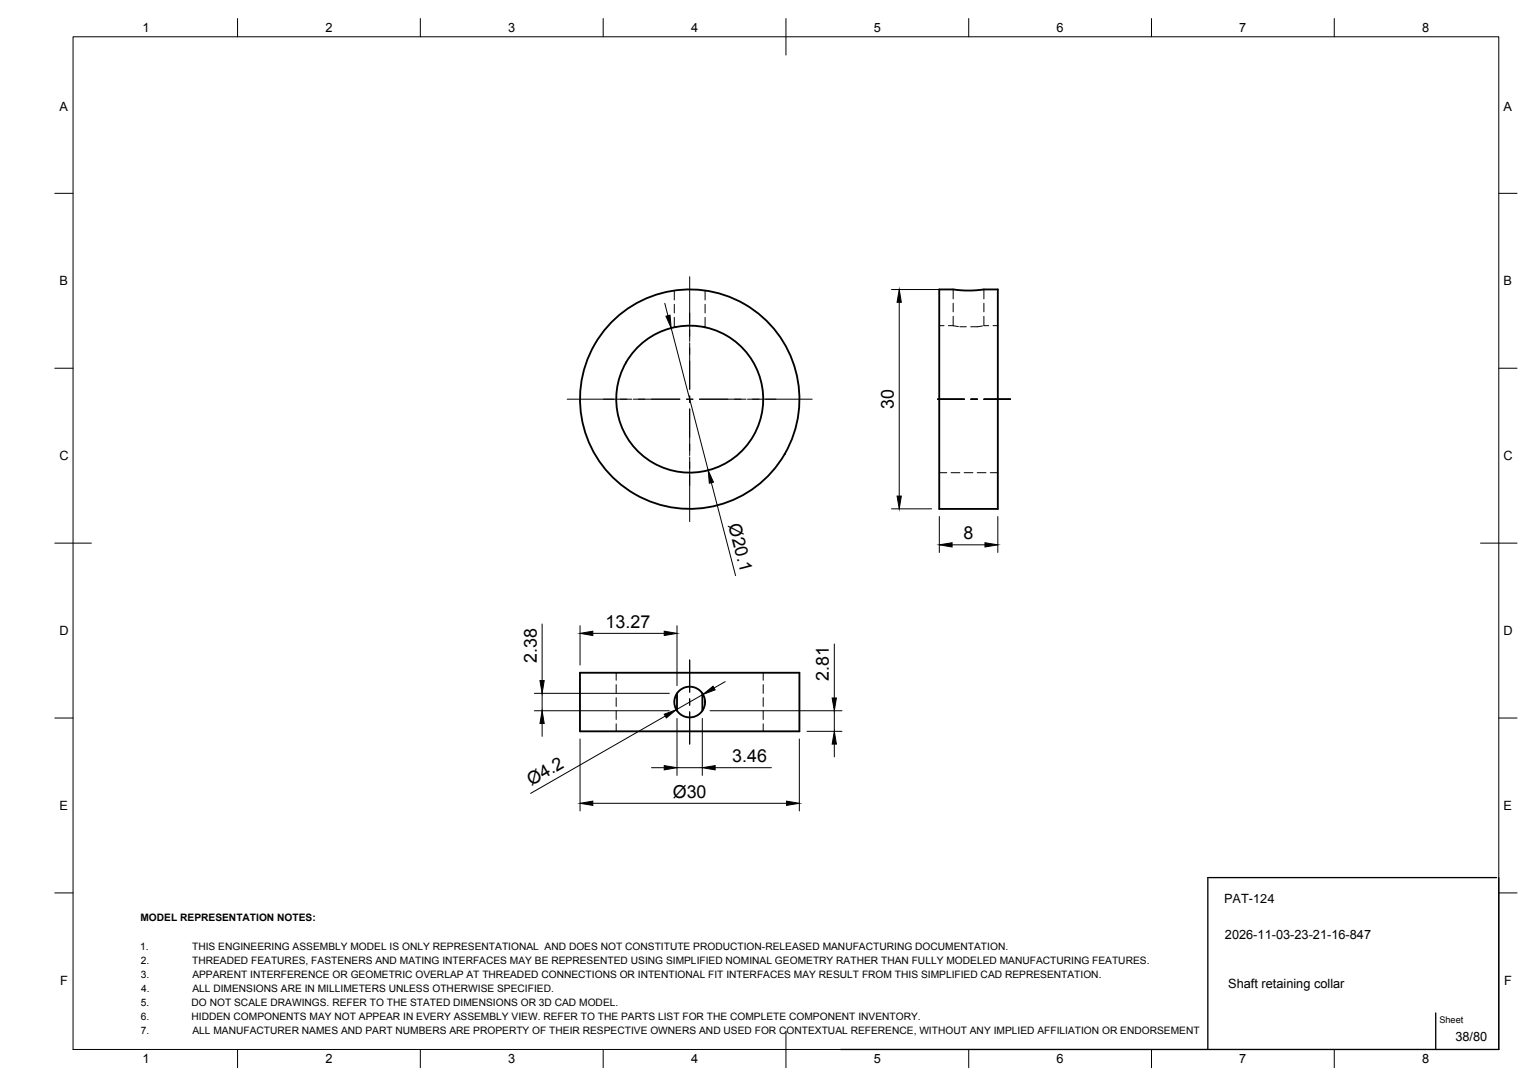
ISO-10303-21;
HEADER;
/* Generated by software containing ST-Developer
 * from STEP Tools, Inc. (www.steptools.com) 
 */

FILE_DESCRIPTION(
/* description */ ('XY cross-slide table'),
/* implementation_level */ '2;1');

FILE_NAME(
/* name */ 'Shaft retaining collar.step',
/* time_stamp */ '2026-10-28T03:22:46-07:00',
/* author */ (''),
/* organization */ (''),
/* preprocessor_version */ 'ST-DEVELOPER v20.2',
/* originating_system */ 'Autodesk Translation Framework v15.17.0.0',
/* authorisation */ '');

FILE_SCHEMA (('AUTOMOTIVE_DESIGN { 1 0 10303 214 3 1 1 }'));
ENDSEC;

DATA;
#10=MECHANICAL_DESIGN_GEOMETRIC_PRESENTATION_REPRESENTATION('',(#1719),#62984);
#1027=B_SPLINE_CURVE_WITH_KNOTS('',3,(#47301,#47302,#47303,#47304,#47305,
#47306,#47307,#47308),.UNSPECIFIED.,.F.,.F.,(4,2,2,4),(0.756005737987019,
0.793568827564653,0.872922520054208,0.952276212543762),.UNSPECIFIED.);
#1028=B_SPLINE_CURVE_WITH_KNOTS('',3,(#47311,#47312,#47313,#47314,#47315,
#47316,#47317,#47318,#47319,#47320,#47321,#47322,#47323,#47324),
 .UNSPECIFIED.,.F.,.F.,(4,2,2,2,2,2,4),(0.121154929624509,0.158718019202145,
0.238071711691699,0.317425404181254,0.396779096670809,0.476132789160363,
0.513695878738001),.UNSPECIFIED.);
#1029=B_SPLINE_CURVE_WITH_KNOTS('',3,(#47325,#47326,#47327,#47328,#47329,
#47330,#47331,#47332),.UNSPECIFIED.,.F.,.F.,(4,2,2,4),(0.952276212543762,
1.03162990503332,1.11098359752287,1.14854668710052),.UNSPECIFIED.);
#1030=B_SPLINE_CURVE_WITH_KNOTS('',3,(#47336,#47337,#47338,#47339,#47340,
#47341,#47342,#47343,#47344,#47345),.UNSPECIFIED.,.F.,.F.,(4,2,2,2,4),(0.,
0.0792165807733642,0.158433161546728,0.237648697074572,0.316864232602417),
 .UNSPECIFIED.);
#1031=B_SPLINE_CURVE_WITH_KNOTS('',3,(#47346,#47347,#47348,#47349,#47350,
#47351,#47352,#47353,#47354,#47355,#47356,#47357,#47358,#47359,#47360,#47361,
#47362,#47363,#47364,#47365,#47366,#47367,#47368,#47369,#47370,#47371),
 .UNSPECIFIED.,.F.,.F.,(4,2,2,2,2,2,2,2,2,2,2,2,4),(0.316864232602417,0.396079768130261,
0.475295303658105,0.554511884431469,0.633728465204833,0.712945045978197,
0.792161626751562,0.871377162279406,0.95059269780725,1.02980823333509,1.10902376886294,
1.1882403496363,1.26745693040967),.UNSPECIFIED.);
#1538=SHAPE_REPRESENTATION_RELATIONSHIP('SRR','None',#63391,#1621);
#1621=ADVANCED_BREP_SHAPE_REPRESENTATION('',(#1829),#62928);
#1719=STYLED_ITEM('',(#63912),#1829);
#1829=MANIFOLD_SOLID_BREP('Body1',#23016);
#2067=FACE_BOUND('',#4939,.T.);
#2068=FACE_BOUND('',#4941,.T.);
#2069=FACE_BOUND('',#4943,.T.);
#2070=FACE_BOUND('',#4945,.T.);
#2529=PLANE('',#25035);
#2530=PLANE('',#25039);
#2531=PLANE('',#25046);
#2532=PLANE('',#25047);
#3441=FACE_OUTER_BOUND('',#4935,.T.);
#3442=FACE_OUTER_BOUND('',#4936,.T.);
#3443=FACE_OUTER_BOUND('',#4937,.T.);
#3444=FACE_OUTER_BOUND('',#4938,.T.);
#3445=FACE_OUTER_BOUND('',#4940,.T.);
#3446=FACE_OUTER_BOUND('',#4942,.T.);
#3447=FACE_OUTER_BOUND('',#4944,.T.);
#4935=EDGE_LOOP('',(#17632,#17633));
#4936=EDGE_LOOP('',(#17634,#17635,#17636,#17637,#17638,#17639,#17640,#17641,
#17642));
#4937=EDGE_LOOP('',(#17643,#17644));
#4938=EDGE_LOOP('',(#17645,#17646,#17647,#17648));
#4939=EDGE_LOOP('',(#17649,#17650,#17651,#17652,#17653));
#4940=EDGE_LOOP('',(#17654,#17655,#17656,#17657));
#4941=EDGE_LOOP('',(#17658,#17659));
#4942=EDGE_LOOP('',(#17660));
#4943=EDGE_LOOP('',(#17661));
#4944=EDGE_LOOP('',(#17662));
#4945=EDGE_LOOP('',(#17663));
#6545=LINE('',#47296,#8032);
#6546=LINE('',#47334,#8033);
#6547=LINE('',#47373,#8034);
#6548=LINE('',#47378,#8035);
#6549=LINE('',#47384,#8036);
#8032=VECTOR('',#29172,1.);
#8033=VECTOR('',#29179,0.210000000000001);
#8034=VECTOR('',#29182,1.);
#8035=VECTOR('',#29187,1.005);
#8036=VECTOR('',#29194,1.5);
#9271=CIRCLE('',#25036,0.210000000000001);
#9272=CIRCLE('',#25038,0.210000000000001);
#9273=CIRCLE('',#25041,1.005);
#9274=CIRCLE('',#25042,1.005);
#9275=CIRCLE('',#25044,1.5);
#9276=CIRCLE('',#25045,1.5);
#10693=VERTEX_POINT('',#47294);
#10694=VERTEX_POINT('',#47295);
#10695=VERTEX_POINT('',#47299);
#10696=VERTEX_POINT('',#47300);
#10697=VERTEX_POINT('',#47309);
#10698=VERTEX_POINT('',#47333);
#10699=VERTEX_POINT('',#47335);
#10700=VERTEX_POINT('',#47375);
#10701=VERTEX_POINT('',#47377);
#10702=VERTEX_POINT('',#47381);
#10703=VERTEX_POINT('',#47383);
#13200=EDGE_CURVE('',#10693,#10694,#6545,.T.);
#13201=EDGE_CURVE('',#10693,#10694,#9271,.T.);
#13202=EDGE_CURVE('',#10695,#10696,#1027,.T.);
#13203=EDGE_CURVE('',#10697,#10695,#9272,.T.);
#13204=EDGE_CURVE('',#10694,#10697,#1028,.T.);
#13205=EDGE_CURVE('',#10696,#10693,#1029,.T.);
#13206=EDGE_CURVE('',#10696,#10698,#6546,.T.);
#13207=EDGE_CURVE('',#10699,#10698,#1030,.T.);
#13208=EDGE_CURVE('',#10698,#10699,#1031,.T.);
#13209=EDGE_CURVE('',#10697,#10695,#6547,.T.);
#13210=EDGE_CURVE('',#10700,#10700,#9273,.T.);
#13211=EDGE_CURVE('',#10700,#10701,#6548,.T.);
#13212=EDGE_CURVE('',#10701,#10701,#9274,.T.);
#13213=EDGE_CURVE('',#10702,#10702,#9275,.T.);
#13214=EDGE_CURVE('',#10702,#10703,#6549,.T.);
#13215=EDGE_CURVE('',#10703,#10703,#9276,.T.);
#17632=ORIENTED_EDGE('',*,*,#13200,.F.);
#17633=ORIENTED_EDGE('',*,*,#13201,.T.);
#17634=ORIENTED_EDGE('',*,*,#13202,.F.);
#17635=ORIENTED_EDGE('',*,*,#13203,.F.);
#17636=ORIENTED_EDGE('',*,*,#13204,.F.);
#17637=ORIENTED_EDGE('',*,*,#13201,.F.);
#17638=ORIENTED_EDGE('',*,*,#13205,.F.);
#17639=ORIENTED_EDGE('',*,*,#13206,.T.);
#17640=ORIENTED_EDGE('',*,*,#13207,.F.);
#17641=ORIENTED_EDGE('',*,*,#13208,.F.);
#17642=ORIENTED_EDGE('',*,*,#13206,.F.);
#17643=ORIENTED_EDGE('',*,*,#13209,.F.);
#17644=ORIENTED_EDGE('',*,*,#13203,.T.);
#17645=ORIENTED_EDGE('',*,*,#13210,.F.);
#17646=ORIENTED_EDGE('',*,*,#13211,.T.);
#17647=ORIENTED_EDGE('',*,*,#13212,.T.);
#17648=ORIENTED_EDGE('',*,*,#13211,.F.);
#17649=ORIENTED_EDGE('',*,*,#13204,.T.);
#17650=ORIENTED_EDGE('',*,*,#13209,.T.);
#17651=ORIENTED_EDGE('',*,*,#13202,.T.);
#17652=ORIENTED_EDGE('',*,*,#13205,.T.);
#17653=ORIENTED_EDGE('',*,*,#13200,.T.);
#17654=ORIENTED_EDGE('',*,*,#13213,.F.);
#17655=ORIENTED_EDGE('',*,*,#13214,.T.);
#17656=ORIENTED_EDGE('',*,*,#13215,.T.);
#17657=ORIENTED_EDGE('',*,*,#13214,.F.);
#17658=ORIENTED_EDGE('',*,*,#13207,.T.);
#17659=ORIENTED_EDGE('',*,*,#13208,.T.);
#17660=ORIENTED_EDGE('',*,*,#13213,.T.);
#17661=ORIENTED_EDGE('',*,*,#13210,.T.);
#17662=ORIENTED_EDGE('',*,*,#13215,.F.);
#17663=ORIENTED_EDGE('',*,*,#13212,.F.);
#21321=CYLINDRICAL_SURFACE('',#25037,0.210000000000001);
#21322=CYLINDRICAL_SURFACE('',#25040,1.005);
#21323=CYLINDRICAL_SURFACE('',#25043,1.5);
#22222=ADVANCED_FACE('',(#3441),#2529,.T.);
#22223=ADVANCED_FACE('',(#3442),#21321,.F.);
#22224=ADVANCED_FACE('',(#3443),#2530,.T.);
#22225=ADVANCED_FACE('',(#3444,#2067),#21322,.F.);
#22226=ADVANCED_FACE('',(#3445,#2068),#21323,.T.);
#22227=ADVANCED_FACE('',(#3446,#2069),#2531,.T.);
#22228=ADVANCED_FACE('',(#3447,#2070),#2532,.F.);
#23016=CLOSED_SHELL('',(#22222,#22223,#22224,#22225,#22226,#22227,#22228));
#25034=AXIS2_PLACEMENT_3D('',#47292,#29168,#29169);
#25035=AXIS2_PLACEMENT_3D('',#47293,#29170,#29171);
#25036=AXIS2_PLACEMENT_3D('',#47297,#29173,#29174);
#25037=AXIS2_PLACEMENT_3D('',#47298,#29175,#29176);
#25038=AXIS2_PLACEMENT_3D('',#47310,#29177,#29178);
#25039=AXIS2_PLACEMENT_3D('',#47372,#29180,#29181);
#25040=AXIS2_PLACEMENT_3D('',#47374,#29183,#29184);
#25041=AXIS2_PLACEMENT_3D('',#47376,#29185,#29186);
#25042=AXIS2_PLACEMENT_3D('',#47379,#29188,#29189);
#25043=AXIS2_PLACEMENT_3D('',#47380,#29190,#29191);
#25044=AXIS2_PLACEMENT_3D('',#47382,#29192,#29193);
#25045=AXIS2_PLACEMENT_3D('',#47385,#29195,#29196);
#25046=AXIS2_PLACEMENT_3D('',#47386,#29197,#29198);
#25047=AXIS2_PLACEMENT_3D('',#47387,#29199,#29200);
#29168=DIRECTION('axis',(0.,0.,1.));
#29169=DIRECTION('refdir',(1.,0.,0.));
#29170=DIRECTION('center_axis',(0.,1.,0.));
#29171=DIRECTION('ref_axis',(1.,0.,0.));
#29172=DIRECTION('',(1.,0.,0.));
#29173=DIRECTION('center_axis',(0.,1.,0.));
#29174=DIRECTION('ref_axis',(1.,0.,0.));
#29175=DIRECTION('center_axis',(0.,1.,0.));
#29176=DIRECTION('ref_axis',(1.,0.,0.));
#29177=DIRECTION('center_axis',(0.,1.,0.));
#29178=DIRECTION('ref_axis',(1.,0.,0.));
#29179=DIRECTION('',(0.,1.,0.));
#29180=DIRECTION('center_axis',(0.,1.,0.));
#29181=DIRECTION('ref_axis',(1.,0.,0.));
#29182=DIRECTION('',(-1.,0.,0.));
#29183=DIRECTION('center_axis',(1.,0.,0.));
#29184=DIRECTION('ref_axis',(0.,0.,-1.));
#29185=DIRECTION('center_axis',(-1.,0.,0.));
#29186=DIRECTION('ref_axis',(0.,0.,-1.));
#29187=DIRECTION('',(-1.,0.,0.));
#29188=DIRECTION('center_axis',(-1.,0.,0.));
#29189=DIRECTION('ref_axis',(0.,0.,-1.));
#29190=DIRECTION('center_axis',(1.,0.,0.));
#29191=DIRECTION('ref_axis',(0.,0.,-1.));
#29192=DIRECTION('center_axis',(1.,0.,0.));
#29193=DIRECTION('ref_axis',(0.,0.,-1.));
#29194=DIRECTION('',(-1.,0.,0.));
#29195=DIRECTION('center_axis',(1.,0.,0.));
#29196=DIRECTION('ref_axis',(0.,0.,-1.));
#29197=DIRECTION('center_axis',(1.,0.,0.));
#29198=DIRECTION('ref_axis',(0.,0.,-1.));
#29199=DIRECTION('center_axis',(1.,0.,0.));
#29200=DIRECTION('ref_axis',(0.,0.,-1.));
#47292=CARTESIAN_POINT('',(0.,0.,0.));
#47293=CARTESIAN_POINT('Origin',(25.8,0.99,4.));
#47294=CARTESIAN_POINT('',(25.6809411910021,0.99,4.17298843892006));
#47295=CARTESIAN_POINT('',(25.9190588089979,0.99,4.17298843892006));
#47296=CARTESIAN_POINT('',(25.4,0.99,4.17298843892006));
#47297=CARTESIAN_POINT('Origin',(25.8,0.99,4.));
#47298=CARTESIAN_POINT('Origin',(25.8,0.99,4.));
#47299=CARTESIAN_POINT('',(25.6809411910021,0.99,3.82701156107994));
#47300=CARTESIAN_POINT('',(25.59,1.005,4.));
#47301=CARTESIAN_POINT('Ctrl Pts',(25.6809411910021,0.989999999999999,3.82701156107994));
#47302=CARTESIAN_POINT('Ctrl Pts',(25.6701985776047,0.99129192197638,3.83440513468868));
#47303=CARTESIAN_POINT('Ctrl Pts',(25.6603122906273,0.992653949439047,3.84270286127439));
#47304=CARTESIAN_POINT('Ctrl Pts',(25.6329072257467,0.996748084390898,3.87010792615492));
#47305=CARTESIAN_POINT('Ctrl Pts',(25.6167579436671,0.999695893276376,3.89366983224072));
#47306=CARTESIAN_POINT('Ctrl Pts',(25.5953022060351,1.00385029472357,3.94538709536759));
#47307=CARTESIAN_POINT('Ctrl Pts',(25.59,1.005,3.97354876917015));
#47308=CARTESIAN_POINT('Ctrl Pts',(25.59,1.005,4.));
#47309=CARTESIAN_POINT('',(25.9190588089979,0.99,3.82701156107994));
#47310=CARTESIAN_POINT('Origin',(25.8,0.99,4.));
#47311=CARTESIAN_POINT('Ctrl Pts',(25.9190588089979,0.99,4.17298843892006));
#47312=CARTESIAN_POINT('Ctrl Pts',(25.9298014223953,0.991291921976381,4.16559486531132));
#47313=CARTESIAN_POINT('Ctrl Pts',(25.9396877093727,0.992653949439047,4.15729713872561));
#47314=CARTESIAN_POINT('Ctrl Pts',(25.9670927742533,0.996748084390898,4.12989207384508));
#47315=CARTESIAN_POINT('Ctrl Pts',(25.9832420563329,0.999695893276376,4.10633016775929));
#47316=CARTESIAN_POINT('Ctrl Pts',(26.0046977939649,1.00385029472357,4.05461290463241));
#47317=CARTESIAN_POINT('Ctrl Pts',(26.01,1.005,4.02645123082985));
#47318=CARTESIAN_POINT('Ctrl Pts',(26.01,1.005,3.97354876917015));
#47319=CARTESIAN_POINT('Ctrl Pts',(26.0046977939649,1.00385029472357,3.94538709536759));
#47320=CARTESIAN_POINT('Ctrl Pts',(25.9832420563329,0.999695893276376,3.89366983224072));
#47321=CARTESIAN_POINT('Ctrl Pts',(25.9670927742533,0.996748084390898,3.87010792615492));
#47322=CARTESIAN_POINT('Ctrl Pts',(25.9396877093727,0.992653949439047,3.84270286127439));
#47323=CARTESIAN_POINT('Ctrl Pts',(25.9298014223953,0.991291921976381,3.83440513468868));
#47324=CARTESIAN_POINT('Ctrl Pts',(25.9190588089979,0.99,3.82701156107994));
#47325=CARTESIAN_POINT('Ctrl Pts',(25.59,1.005,4.));
#47326=CARTESIAN_POINT('Ctrl Pts',(25.59,1.005,4.02645123082985));
#47327=CARTESIAN_POINT('Ctrl Pts',(25.5953022060351,1.00385029472357,4.05461290463241));
#47328=CARTESIAN_POINT('Ctrl Pts',(25.6167579436671,0.999695893276376,4.10633016775929));
#47329=CARTESIAN_POINT('Ctrl Pts',(25.6329072257467,0.996748084390898,4.12989207384508));
#47330=CARTESIAN_POINT('Ctrl Pts',(25.6603122906273,0.992653949439047,4.15729713872561));
#47331=CARTESIAN_POINT('Ctrl Pts',(25.6701985776047,0.991291921976381,4.16559486531132));
#47332=CARTESIAN_POINT('Ctrl Pts',(25.6809411910021,0.99,4.17298843892006));
#47333=CARTESIAN_POINT('',(25.59,1.5,4.));
#47334=CARTESIAN_POINT('',(25.59,0.99,4.));
#47335=CARTESIAN_POINT('',(25.8,1.48522725533839,4.21));
#47336=CARTESIAN_POINT('Ctrl Pts',(25.8,1.48522725533839,4.21));
#47337=CARTESIAN_POINT('Ctrl Pts',(25.7735944730755,1.48522725533839,4.21));
#47338=CARTESIAN_POINT('Ctrl Pts',(25.7454529259093,1.48600415954412,4.2047157372696));
#47339=CARTESIAN_POINT('Ctrl Pts',(25.6937237310949,1.48880073282317,4.18327376303633));
#47340=CARTESIAN_POINT('Ctrl Pts',(25.670133075872,1.49077897157582,4.16711792397039));
#47341=CARTESIAN_POINT('Ctrl Pts',(25.632882321789,1.49448481141327,4.12986716988737));
#47342=CARTESIAN_POINT('Ctrl Pts',(25.6167262899986,1.49645455657129,4.10627640830577));
#47343=CARTESIAN_POINT('Ctrl Pts',(25.5952841751738,1.49923165515646,4.0545468514059));
#47344=CARTESIAN_POINT('Ctrl Pts',(25.59,1.5,4.02640517850928));
#47345=CARTESIAN_POINT('Ctrl Pts',(25.59,1.5,4.));
#47346=CARTESIAN_POINT('Ctrl Pts',(25.59,1.5,4.));
#47347=CARTESIAN_POINT('Ctrl Pts',(25.59,1.5,3.97359482149072));
#47348=CARTESIAN_POINT('Ctrl Pts',(25.5952841751738,1.49923165515646,3.9454531485941));
#47349=CARTESIAN_POINT('Ctrl Pts',(25.6167262899986,1.49645455657129,3.89372359169423));
#47350=CARTESIAN_POINT('Ctrl Pts',(25.632882321789,1.49448481141327,3.87013283011263));
#47351=CARTESIAN_POINT('Ctrl Pts',(25.670133075872,1.49077897157582,3.83288207602961));
#47352=CARTESIAN_POINT('Ctrl Pts',(25.6937237310949,1.48880073282317,3.81672623696366));
#47353=CARTESIAN_POINT('Ctrl Pts',(25.7454529259093,1.48600415954412,3.7952842627304));
#47354=CARTESIAN_POINT('Ctrl Pts',(25.7735944730755,1.48522725533839,3.79));
#47355=CARTESIAN_POINT('Ctrl Pts',(25.8264055269245,1.48522725533839,3.79));
#47356=CARTESIAN_POINT('Ctrl Pts',(25.8545470740907,1.48600415954412,3.7952842627304));
#47357=CARTESIAN_POINT('Ctrl Pts',(25.9062762689051,1.48880073282317,3.81672623696367));
#47358=CARTESIAN_POINT('Ctrl Pts',(25.929866924128,1.49077897157582,3.83288207602961));
#47359=CARTESIAN_POINT('Ctrl Pts',(25.967117678211,1.49448481141327,3.87013283011263));
#47360=CARTESIAN_POINT('Ctrl Pts',(25.9832737100014,1.49645455657129,3.89372359169423));
#47361=CARTESIAN_POINT('Ctrl Pts',(26.0047158248262,1.49923165515646,3.9454531485941));
#47362=CARTESIAN_POINT('Ctrl Pts',(26.01,1.5,3.97359482149072));
#47363=CARTESIAN_POINT('Ctrl Pts',(26.01,1.5,4.02640517850928));
#47364=CARTESIAN_POINT('Ctrl Pts',(26.0047158248262,1.49923165515646,4.0545468514059));
#47365=CARTESIAN_POINT('Ctrl Pts',(25.9832737100014,1.49645455657129,4.10627640830577));
#47366=CARTESIAN_POINT('Ctrl Pts',(25.967117678211,1.49448481141327,4.12986716988737));
#47367=CARTESIAN_POINT('Ctrl Pts',(25.929866924128,1.49077897157582,4.16711792397039));
#47368=CARTESIAN_POINT('Ctrl Pts',(25.9062762689051,1.48880073282317,4.18327376303633));
#47369=CARTESIAN_POINT('Ctrl Pts',(25.8545470740907,1.48600415954412,4.20471573726959));
#47370=CARTESIAN_POINT('Ctrl Pts',(25.8264055269245,1.48522725533839,4.21));
#47371=CARTESIAN_POINT('Ctrl Pts',(25.8,1.48522725533839,4.21));
#47372=CARTESIAN_POINT('Origin',(25.8,0.99,4.));
#47373=CARTESIAN_POINT('',(25.4,0.99,3.82701156107994));
#47374=CARTESIAN_POINT('Origin',(25.4,0.,4.));
#47375=CARTESIAN_POINT('',(26.2,-1.23077003314309E-16,5.005));
#47376=CARTESIAN_POINT('Origin',(26.2,0.,4.));
#47377=CARTESIAN_POINT('',(25.4,-1.23077003314309E-16,5.005));
#47378=CARTESIAN_POINT('',(25.4,-1.23077003314309E-16,5.005));
#47379=CARTESIAN_POINT('Origin',(25.4,0.,4.));
#47380=CARTESIAN_POINT('Origin',(25.4,0.,4.));
#47381=CARTESIAN_POINT('',(26.2,-1.83697019872103E-16,5.5));
#47382=CARTESIAN_POINT('Origin',(26.2,0.,4.));
#47383=CARTESIAN_POINT('',(25.4,-1.83697019872103E-16,5.5));
#47384=CARTESIAN_POINT('',(25.4,-1.83697019872103E-16,5.5));
#47385=CARTESIAN_POINT('Origin',(25.4,0.,4.));
#47386=CARTESIAN_POINT('Origin',(26.2,0.,4.));
#47387=CARTESIAN_POINT('Origin',(25.4,0.,4.));
#62829=UNCERTAINTY_MEASURE_WITH_UNIT(LENGTH_MEASURE(0.001),#62985,
'DISTANCE_ACCURACY_VALUE',
'Maximum model space distance between geometric entities at asserted c
onnectivities');
#62885=UNCERTAINTY_MEASURE_WITH_UNIT(LENGTH_MEASURE(0.001),#62985,
'DISTANCE_ACCURACY_VALUE',
'Maximum model space distance between geometric entities at asserted c
onnectivities');
#62928=(
GEOMETRIC_REPRESENTATION_CONTEXT(3)
GLOBAL_UNCERTAINTY_ASSIGNED_CONTEXT((#62829))
GLOBAL_UNIT_ASSIGNED_CONTEXT((#62985,#62987,#62988))
REPRESENTATION_CONTEXT('','3D')
);
#62984=(
GEOMETRIC_REPRESENTATION_CONTEXT(3)
GLOBAL_UNCERTAINTY_ASSIGNED_CONTEXT((#62885))
GLOBAL_UNIT_ASSIGNED_CONTEXT((#62985,#62987,#62988))
REPRESENTATION_CONTEXT('','3D')
);
#62985=(
LENGTH_UNIT()
NAMED_UNIT(*)
SI_UNIT(.CENTI.,.METRE.)
);
#62987=(
NAMED_UNIT(*)
PLANE_ANGLE_UNIT()
SI_UNIT($,.RADIAN.)
);
#62988=(
NAMED_UNIT(*)
SI_UNIT($,.STERADIAN.)
SOLID_ANGLE_UNIT()
);
#63031=SHAPE_DEFINITION_REPRESENTATION(#63162,#63391);
#63162=PRODUCT_DEFINITION_SHAPE('',$,#63490);
#63391=SHAPE_REPRESENTATION('',(#25034),#62928);
#63447=PRODUCT_DEFINITION_CONTEXT('part definition',#63743,'design');
#63490=PRODUCT_DEFINITION('Shaft retaining collar',
'Shaft retaining collar',#63588,#63447);
#63588=PRODUCT_DEFINITION_FORMATION('',$,#63787);
#63743=APPLICATION_CONTEXT(
'Core Data for Automotive Mechanical Design Process');
#63744=PRODUCT_CONTEXT('part definition',#63743,'mechanical');
#63787=PRODUCT('Shaft retaining collar','Shaft retaining collar',
'Shaft retaining collar',(#63744));
#63906=COLOUR_RGB('Grey',0.48,0.52,0.57);
#63907=FILL_AREA_STYLE_COLOUR('',#63906);
#63908=FILL_AREA_STYLE('',(#63907));
#63909=SURFACE_STYLE_FILL_AREA(#63908);
#63910=SURFACE_SIDE_STYLE('',(#63909));
#63911=SURFACE_STYLE_USAGE(.BOTH.,#63910);
#63912=PRESENTATION_STYLE_ASSIGNMENT((#63911));
ENDSEC;
END-ISO-10303-21;
